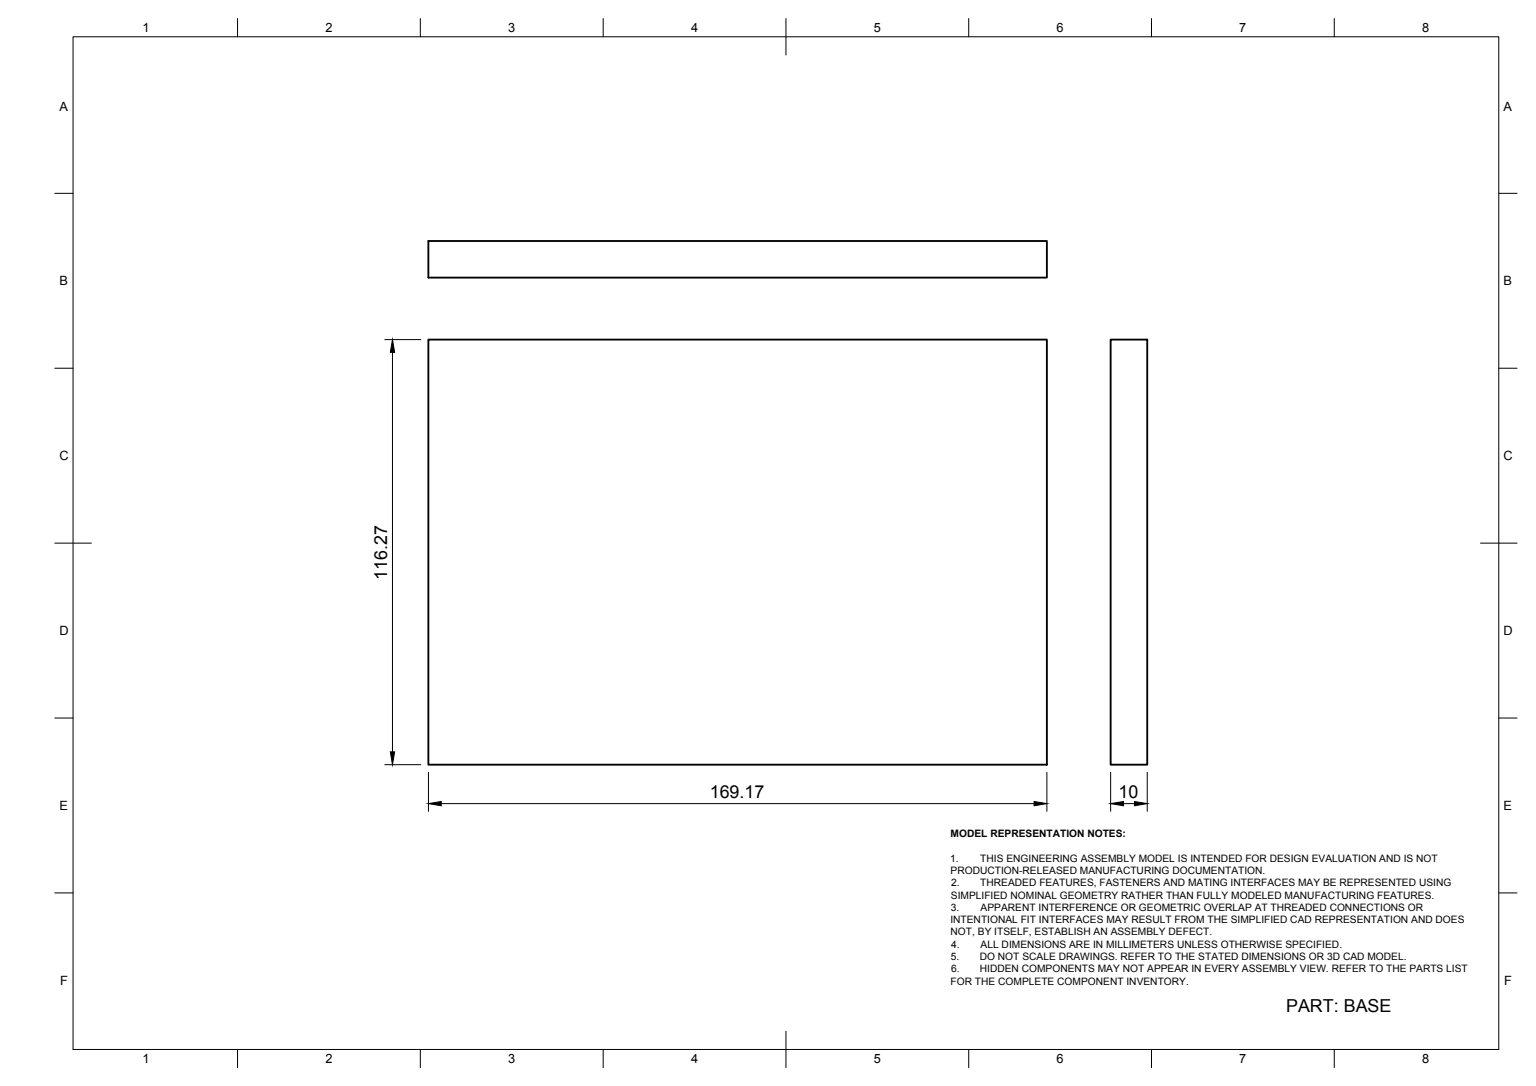
ISO-10303-21;
HEADER;
/* Generated by software containing ST-Developer
 * from STEP Tools, Inc. (www.steptools.com) 
 */

FILE_DESCRIPTION(
/* description */ (''),
/* implementation_level */ '2;1');

FILE_NAME(
/* name */ 'Base.step',
/* time_stamp */ '2026-09-20T22:38:01+06:00',
/* author */ (''),
/* organization */ (''),
/* preprocessor_version */ 'ST-DEVELOPER v20.2',
/* originating_system */ 'Autodesk Translation Framework v15.15.0.0',
/* authorisation */ '');

FILE_SCHEMA (('AUTOMOTIVE_DESIGN { 1 0 10303 214 3 1 1 }'));
ENDSEC;

DATA;
#10=MECHANICAL_DESIGN_GEOMETRIC_PRESENTATION_REPRESENTATION('',(#90),#4079);
#74=SHAPE_REPRESENTATION_RELATIONSHIP('SRR','None',#4117,#82);
#82=ADVANCED_BREP_SHAPE_REPRESENTATION('',(#98),#4077);
#90=STYLED_ITEM('',(#4159),#98);
#98=MANIFOLD_SOLID_BREP('Base',#1449);
#272=FACE_OUTER_BOUND('',#362,.T.);
#273=FACE_OUTER_BOUND('',#363,.T.);
#274=FACE_OUTER_BOUND('',#364,.T.);
#275=FACE_OUTER_BOUND('',#365,.T.);
#276=FACE_OUTER_BOUND('',#366,.T.);
#277=FACE_OUTER_BOUND('',#367,.T.);
#362=EDGE_LOOP('',(#1279,#1280,#1281,#1282));
#363=EDGE_LOOP('',(#1283,#1284,#1285,#1286));
#364=EDGE_LOOP('',(#1287,#1288,#1289,#1290));
#365=EDGE_LOOP('',(#1291,#1292,#1293,#1294));
#366=EDGE_LOOP('',(#1295,#1296,#1297,#1298));
#367=EDGE_LOOP('',(#1299,#1300,#1301,#1302));
#471=LINE('',#4020,#584);
#472=LINE('',#4022,#585);
#473=LINE('',#4024,#586);
#474=LINE('',#4025,#587);
#475=LINE('',#4028,#588);
#476=LINE('',#4030,#589);
#477=LINE('',#4031,#590);
#478=LINE('',#4034,#591);
#479=LINE('',#4036,#592);
#480=LINE('',#4037,#593);
#481=LINE('',#4039,#594);
#482=LINE('',#4040,#595);
#584=VECTOR('',#2076,10.);
#585=VECTOR('',#2077,10.);
#586=VECTOR('',#2078,10.);
#587=VECTOR('',#2079,10.);
#588=VECTOR('',#2082,10.);
#589=VECTOR('',#2083,10.);
#590=VECTOR('',#2084,10.);
#591=VECTOR('',#2087,10.);
#592=VECTOR('',#2088,10.);
#593=VECTOR('',#2089,10.);
#594=VECTOR('',#2092,10.);
#595=VECTOR('',#2093,10.);
#714=VERTEX_POINT('',#4018);
#715=VERTEX_POINT('',#4019);
#716=VERTEX_POINT('',#4021);
#717=VERTEX_POINT('',#4023);
#718=VERTEX_POINT('',#4027);
#719=VERTEX_POINT('',#4029);
#720=VERTEX_POINT('',#4033);
#721=VERTEX_POINT('',#4035);
#904=EDGE_CURVE('',#714,#715,#471,.T.);
#905=EDGE_CURVE('',#714,#716,#472,.T.);
#906=EDGE_CURVE('',#717,#716,#473,.T.);
#907=EDGE_CURVE('',#715,#717,#474,.T.);
#908=EDGE_CURVE('',#715,#718,#475,.T.);
#909=EDGE_CURVE('',#719,#717,#476,.T.);
#910=EDGE_CURVE('',#718,#719,#477,.T.);
#911=EDGE_CURVE('',#718,#720,#478,.T.);
#912=EDGE_CURVE('',#721,#719,#479,.T.);
#913=EDGE_CURVE('',#720,#721,#480,.T.);
#914=EDGE_CURVE('',#720,#714,#481,.T.);
#915=EDGE_CURVE('',#716,#721,#482,.T.);
#1279=ORIENTED_EDGE('',*,*,#904,.F.);
#1280=ORIENTED_EDGE('',*,*,#905,.T.);
#1281=ORIENTED_EDGE('',*,*,#906,.F.);
#1282=ORIENTED_EDGE('',*,*,#907,.F.);
#1283=ORIENTED_EDGE('',*,*,#908,.F.);
#1284=ORIENTED_EDGE('',*,*,#907,.T.);
#1285=ORIENTED_EDGE('',*,*,#909,.F.);
#1286=ORIENTED_EDGE('',*,*,#910,.F.);
#1287=ORIENTED_EDGE('',*,*,#911,.F.);
#1288=ORIENTED_EDGE('',*,*,#910,.T.);
#1289=ORIENTED_EDGE('',*,*,#912,.F.);
#1290=ORIENTED_EDGE('',*,*,#913,.F.);
#1291=ORIENTED_EDGE('',*,*,#914,.F.);
#1292=ORIENTED_EDGE('',*,*,#913,.T.);
#1293=ORIENTED_EDGE('',*,*,#915,.F.);
#1294=ORIENTED_EDGE('',*,*,#905,.F.);
#1295=ORIENTED_EDGE('',*,*,#915,.T.);
#1296=ORIENTED_EDGE('',*,*,#912,.T.);
#1297=ORIENTED_EDGE('',*,*,#909,.T.);
#1298=ORIENTED_EDGE('',*,*,#906,.T.);
#1299=ORIENTED_EDGE('',*,*,#914,.T.);
#1300=ORIENTED_EDGE('',*,*,#904,.T.);
#1301=ORIENTED_EDGE('',*,*,#908,.T.);
#1302=ORIENTED_EDGE('',*,*,#911,.T.);
#1351=PLANE('',#1678);
#1352=PLANE('',#1679);
#1353=PLANE('',#1680);
#1354=PLANE('',#1681);
#1355=PLANE('',#1682);
#1356=PLANE('',#1683);
#1434=ADVANCED_FACE('',(#272),#1351,.T.);
#1435=ADVANCED_FACE('',(#273),#1352,.T.);
#1436=ADVANCED_FACE('',(#274),#1353,.T.);
#1437=ADVANCED_FACE('',(#275),#1354,.T.);
#1438=ADVANCED_FACE('',(#276),#1355,.T.);
#1439=ADVANCED_FACE('',(#277),#1356,.F.);
#1449=CLOSED_SHELL('',(#1434,#1435,#1436,#1437,#1438,#1439));
#1677=AXIS2_PLACEMENT_3D('',#4016,#2072,#2073);
#1678=AXIS2_PLACEMENT_3D('',#4017,#2074,#2075);
#1679=AXIS2_PLACEMENT_3D('',#4026,#2080,#2081);
#1680=AXIS2_PLACEMENT_3D('',#4032,#2085,#2086);
#1681=AXIS2_PLACEMENT_3D('',#4038,#2090,#2091);
#1682=AXIS2_PLACEMENT_3D('',#4041,#2094,#2095);
#1683=AXIS2_PLACEMENT_3D('',#4042,#2096,#2097);
#2072=DIRECTION('axis',(0.,0.,1.));
#2073=DIRECTION('refdir',(1.,0.,0.));
#2074=DIRECTION('center_axis',(1.,0.,0.));
#2075=DIRECTION('ref_axis',(0.,0.,-1.));
#2076=DIRECTION('',(0.,0.,1.));
#2077=DIRECTION('',(0.,1.,0.));
#2078=DIRECTION('',(0.,0.,-1.));
#2079=DIRECTION('',(0.,1.,0.));
#2080=DIRECTION('center_axis',(0.,0.,1.));
#2081=DIRECTION('ref_axis',(1.,0.,0.));
#2082=DIRECTION('',(-1.,0.,0.));
#2083=DIRECTION('',(1.,0.,0.));
#2084=DIRECTION('',(0.,1.,0.));
#2085=DIRECTION('center_axis',(-1.,0.,0.));
#2086=DIRECTION('ref_axis',(0.,0.,1.));
#2087=DIRECTION('',(0.,0.,-1.));
#2088=DIRECTION('',(0.,0.,1.));
#2089=DIRECTION('',(0.,1.,0.));
#2090=DIRECTION('center_axis',(0.,0.,-1.));
#2091=DIRECTION('ref_axis',(-1.,0.,0.));
#2092=DIRECTION('',(1.,0.,0.));
#2093=DIRECTION('',(-1.,0.,0.));
#2094=DIRECTION('center_axis',(0.,1.,0.));
#2095=DIRECTION('ref_axis',(0.,0.,1.));
#2096=DIRECTION('center_axis',(0.,1.,0.));
#2097=DIRECTION('ref_axis',(1.,0.,0.));
#4016=CARTESIAN_POINT('',(0.,0.,0.));
#4017=CARTESIAN_POINT('Origin',(101.305059905209,5.,116.266583003001));
#4018=CARTESIAN_POINT('',(101.305059905209,5.,0.));
#4019=CARTESIAN_POINT('',(101.305059905209,5.,116.266583003001));
#4020=CARTESIAN_POINT('',(101.305059905209,5.,0.));
#4021=CARTESIAN_POINT('',(101.305059905209,15.,0.));
#4022=CARTESIAN_POINT('',(101.305059905209,5.,0.));
#4023=CARTESIAN_POINT('',(101.305059905209,15.,116.266583003001));
#4024=CARTESIAN_POINT('',(101.305059905209,15.,0.));
#4025=CARTESIAN_POINT('',(101.305059905209,5.,116.266583003001));
#4026=CARTESIAN_POINT('Origin',(-67.8619652977995,5.,116.266583003001));
#4027=CARTESIAN_POINT('',(-67.8619652977995,5.,116.266583003001));
#4028=CARTESIAN_POINT('',(101.305059905209,5.,116.266583003001));
#4029=CARTESIAN_POINT('',(-67.8619652977995,15.,116.266583003001));
#4030=CARTESIAN_POINT('',(101.305059905209,15.,116.266583003001));
#4031=CARTESIAN_POINT('',(-67.8619652977995,5.,116.266583003001));
#4032=CARTESIAN_POINT('Origin',(-67.8619652977995,5.,0.));
#4033=CARTESIAN_POINT('',(-67.8619652977995,5.,0.));
#4034=CARTESIAN_POINT('',(-67.8619652977995,5.,116.266583003001));
#4035=CARTESIAN_POINT('',(-67.8619652977995,15.,0.));
#4036=CARTESIAN_POINT('',(-67.8619652977995,15.,116.266583003001));
#4037=CARTESIAN_POINT('',(-67.8619652977995,5.,0.));
#4038=CARTESIAN_POINT('Origin',(101.305059905209,5.,0.));
#4039=CARTESIAN_POINT('',(-67.8619652977995,5.,0.));
#4040=CARTESIAN_POINT('',(-67.8619652977995,15.,0.));
#4041=CARTESIAN_POINT('Origin',(16.721547303705,15.,58.1332915015007));
#4042=CARTESIAN_POINT('Origin',(16.721547303705,5.,58.1332915015007));
#4067=UNCERTAINTY_MEASURE_WITH_UNIT(LENGTH_MEASURE(0.01),#4080,
'DISTANCE_ACCURACY_VALUE',
'Maximum model space distance between geometric entities at asserted c
onnectivities');
#4069=UNCERTAINTY_MEASURE_WITH_UNIT(LENGTH_MEASURE(0.01),#4080,
'DISTANCE_ACCURACY_VALUE',
'Maximum model space distance between geometric entities at asserted c
onnectivities');
#4077=(
GEOMETRIC_REPRESENTATION_CONTEXT(3)
GLOBAL_UNCERTAINTY_ASSIGNED_CONTEXT((#4067))
GLOBAL_UNIT_ASSIGNED_CONTEXT((#4080,#4082,#4083))
REPRESENTATION_CONTEXT('','3D')
);
#4079=(
GEOMETRIC_REPRESENTATION_CONTEXT(3)
GLOBAL_UNCERTAINTY_ASSIGNED_CONTEXT((#4069))
GLOBAL_UNIT_ASSIGNED_CONTEXT((#4080,#4082,#4083))
REPRESENTATION_CONTEXT('','3D')
);
#4080=(
LENGTH_UNIT()
NAMED_UNIT(*)
SI_UNIT(.MILLI.,.METRE.)
);
#4082=(
NAMED_UNIT(*)
PLANE_ANGLE_UNIT()
SI_UNIT($,.RADIAN.)
);
#4083=(
NAMED_UNIT(*)
SI_UNIT($,.STERADIAN.)
SOLID_ANGLE_UNIT()
);
#4091=SHAPE_DEFINITION_REPRESENTATION(#4100,#4117);
#4100=PRODUCT_DEFINITION_SHAPE('',$,#4127);
#4117=SHAPE_REPRESENTATION('',(#1677),#4077);
#4119=PRODUCT_DEFINITION_CONTEXT('part definition',#4148,'design');
#4127=PRODUCT_DEFINITION('Base','Base',#4136,#4119);
#4136=PRODUCT_DEFINITION_FORMATION('',$,#4157);
#4148=APPLICATION_CONTEXT(
'Core Data for Automotive Mechanical Design Process');
#4149=PRODUCT_CONTEXT('part definition',#4148,'mechanical');
#4157=PRODUCT('Base','Base',$,(#4149));
#4159=PRESENTATION_STYLE_ASSIGNMENT((#4163));
#4163=SURFACE_STYLE_USAGE(.BOTH.,#4167);
#4167=SURFACE_SIDE_STYLE('',(#4171));
#4171=SURFACE_STYLE_FILL_AREA(#4175);
#4175=FILL_AREA_STYLE('Steel - Satin',(#4179));
#4179=FILL_AREA_STYLE_COLOUR('Steel - Satin',#4183);
#4183=COLOUR_RGB('Steel - Satin', 0.40784314, 0.44705882, 0.49803922);
ENDSEC;
END-ISO-10303-21;
